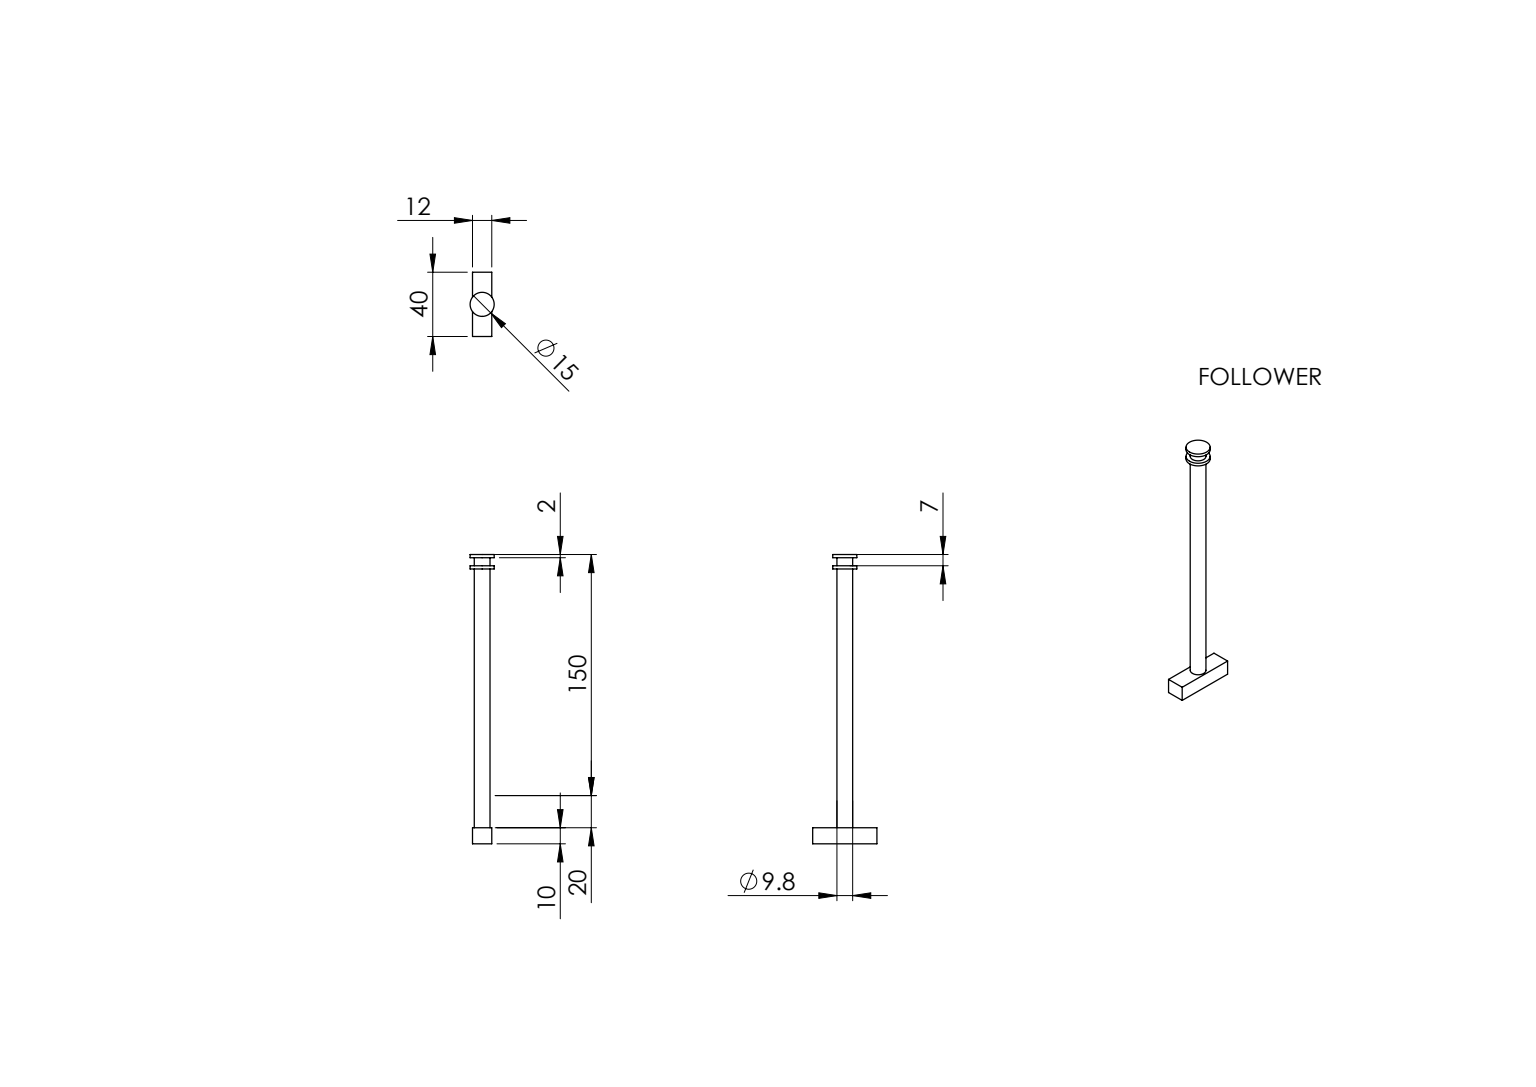
ISO-10303-21;
HEADER;
FILE_DESCRIPTION (('STEP AP214'),
    '1' );
FILE_NAME ('follower.step',
    '2026-10-31T03:36:27',
    ( '' ),
    ( '' ),
    'SwSTEP 2.0',
    'SolidWorks 2026',
    '' );
FILE_SCHEMA (( 'AUTOMOTIVE_DESIGN' ));
ENDSEC;

DATA;
#15=ORIENTED_EDGE ( 'NONE', *, *, #13669, .F. ) ;
#100=DIRECTION ( 'NONE',  ( -1.000000000000000000, 0.000000000000000000, 5.782411586589356653E-16 ) ) ;
#105=AXIS2_PLACEMENT_3D ( 'NONE', #31796, #37295, #28576 ) ;
#107=LINE ( 'NONE', #3514, #14620 ) ;
#160=UNCERTAINTY_MEASURE_WITH_UNIT (LENGTH_MEASURE( 1.000000000000000082E-05 ), #19760, 'distance_accuracy_value', 'NONE');
#194=CARTESIAN_POINT ( 'NONE',  ( 5.999999999999999112, -30.00000000000000000, -19.99999999999999289 ) ) ;
#273=FACE_OUTER_BOUND ( 'NONE', #13038, .T. ) ;
#337=AXIS2_PLACEMENT_3D ( 'NONE', #15365, #24083, #35628 ) ;
#423=CARTESIAN_POINT ( 'NONE',  ( 0.000000000000000000, 143.0000000000000000, 0.000000000000000000 ) ) ;
#429=ORIENTED_EDGE ( 'NONE', *, *, #547, .F. ) ;
#505=EDGE_LOOP ( 'NONE', ( #36598, #28782, #25690, #21960 ) ) ;
#547=EDGE_CURVE ( 'NONE', #14469, #8607, #31068, .T. ) ;
#642=CYLINDRICAL_SURFACE ( 'NONE', #12591, 4.899999999999999467 ) ;
#732=LINE ( 'NONE', #35796, #24881 ) ;
#762=VERTEX_POINT ( 'NONE', #1446 ) ;
#937=AXIS2_PLACEMENT_3D ( 'NONE', #24457, #33914, #7396 ) ;
#980=ORIENTED_EDGE ( 'NONE', *, *, #3451, .T. ) ;
#1025=ORIENTED_EDGE ( 'NONE', *, *, #37375, .T. ) ;
#1100=VECTOR ( 'NONE', #32793, 1000.000000000000000 ) ;
#1108=PLANE ( 'NONE',  #11917 ) ;
#1181=ORIENTED_EDGE ( 'NONE', *, *, #19610, .T. ) ;
#1231=ORIENTED_EDGE ( 'NONE', *, *, #34414, .F. ) ;
#1293=ADVANCED_FACE ( 'NONE', ( #273 ), #642, .T. ) ;
#1351=VERTEX_POINT ( 'NONE', #6531 ) ;
#1446=CARTESIAN_POINT ( 'NONE',  ( -6.000000000000000888, -30.00000000000000000, 20.00000000000000711 ) ) ;
#1468=LINE ( 'NONE', #22824, #18170 ) ;
#1631=SHAPE_DEFINITION_REPRESENTATION ( #19546, #8404 ) ;
#1734=VECTOR ( 'NONE', #11519, 1000.000000000000000 ) ;
#1890=ORIENTED_EDGE ( 'NONE', *, *, #32981, .F. ) ;
#2042=AXIS2_PLACEMENT_3D ( 'NONE', #31159, #28304, #16756 ) ;
#2104=CARTESIAN_POINT ( 'NONE',  ( 0.000000000000000000, 150.0000000000000000, 0.000000000000000000 ) ) ;
#2125=ORIENTED_EDGE ( 'NONE', *, *, #27701, .F. ) ;
#2222=EDGE_CURVE ( 'NONE', #13040, #5701, #9847, .T. ) ;
#2244=DIRECTION ( 'NONE',  ( 0.000000000000000000, 0.000000000000000000, 1.000000000000000000 ) ) ;
#2290=DIRECTION ( 'NONE',  ( 0.000000000000000000, -0.000000000000000000, 1.000000000000000000 ) ) ;
#2448=MECHANICAL_DESIGN_GEOMETRIC_PRESENTATION_REPRESENTATION('',(#13958),#24243);
#2589=DIRECTION ( 'NONE',  ( 0.000000000000000000, 0.000000000000000000, 1.000000000000000000 ) ) ;
#2592=ORIENTED_EDGE ( 'NONE', *, *, #17340, .F. ) ;
#2619=ORIENTED_EDGE ( 'NONE', *, *, #17340, .T. ) ;
#2703=PLANE ( 'NONE',  #2042 ) ;
#2990=CARTESIAN_POINT ( 'NONE',  ( 6.000000000000000000, -30.00000000000000000, 20.00000000000000000 ) ) ;
#3152=PRODUCT_DEFINITION_CONTEXT ( 'detailed design', #6891, 'design' ) ;
#3165=ORIENTED_EDGE ( 'NONE', *, *, #32431, .T. ) ;
#3269=CARTESIAN_POINT ( 'NONE',  ( 5.999999999999999112, -20.00000000000000000, -19.99999999999999289 ) ) ;
#3315=ADVANCED_FACE ( 'NONE', ( #19149 ), #27843, .T. ) ;
#3355=ORIENTED_EDGE ( 'NONE', *, *, #23085, .F. ) ;
#3361=ORIENTED_EDGE ( 'NONE', *, *, #26146, .F. ) ;
#3451=EDGE_CURVE ( 'NONE', #34986, #25827, #27661, .T. ) ;
#3459=EDGE_CURVE ( 'NONE', #4369, #32041, #34461, .T. ) ;
#3496=APPLICATION_CONTEXT ( 'automotive_design' ) ;
#3514=CARTESIAN_POINT ( 'NONE',  ( 6.000769315822030740E-16, -20.00000000000000000, -4.899999999999999467 ) ) ;
#3572=EDGE_CURVE ( 'NONE', #1351, #25827, #28567, .T. ) ;
#3716=DIRECTION ( 'NONE',  ( -1.000000000000000000, -0.000000000000000000, 5.782411586589356653E-16 ) ) ;
#3876=DIRECTION ( 'NONE',  ( 0.000000000000000000, 1.000000000000000000, 0.000000000000000000 ) ) ;
#3931=CARTESIAN_POINT ( 'NONE',  ( 0.000000000000000000, -20.00000000000000000, 0.000000000000000000 ) ) ;
#4270=EDGE_LOOP ( 'NONE', ( #13366, #36759, #31537, #32986 ) ) ;
#4310=ORIENTED_EDGE ( 'NONE', *, *, #8311, .F. ) ;
#4369=VERTEX_POINT ( 'NONE', #27616 ) ;
#4439=CARTESIAN_POINT ( 'NONE',  ( 0.000000000000000000, -20.00000000000000000, 4.899999999999999467 ) ) ;
#4528=DIRECTION ( 'NONE',  ( -0.000000000000000000, -1.000000000000000000, -0.000000000000000000 ) ) ;
#4534=DIRECTION ( 'NONE',  ( 0.000000000000000000, 1.000000000000000000, 0.000000000000000000 ) ) ;
#4651=DIRECTION ( 'NONE',  ( 0.000000000000000000, 0.000000000000000000, 1.000000000000000000 ) ) ;
#4744=CLOSED_SHELL ( 'NONE', ( #24245, #27494, #28200, #19192, #1293, #6469, #32100, #16308, #5411, #18285, #28238, #3315, #20115, #18072, #18295, #24769, #16663, #12725 ) ) ;
#4791=DIRECTION ( 'NONE',  ( 1.000000000000000000, 0.000000000000000000, -0.000000000000000000 ) ) ;
#4965=EDGE_CURVE ( 'NONE', #23915, #23913, #20695, .T. ) ;
#5029=AXIS2_PLACEMENT_3D ( 'NONE', #14926, #6766, #29888 ) ;
#5066=ORIENTED_EDGE ( 'NONE', *, *, #29640, .T. ) ;
#5156=AXIS2_PLACEMENT_3D ( 'NONE', #20310, #31851, #28999 ) ;
#5411=ADVANCED_FACE ( 'NONE', ( #19800 ), #2703, .F. ) ;
#5574=( NAMED_UNIT ( * ) SI_UNIT ( $, .STERADIAN. ) SOLID_ANGLE_UNIT ( ) );
#5638=( GEOMETRIC_REPRESENTATION_CONTEXT ( 3 ) GLOBAL_UNCERTAINTY_ASSIGNED_CONTEXT ( ( #13508 ) ) GLOBAL_UNIT_ASSIGNED_CONTEXT ( ( #28887, #11461, #29253 ) ) REPRESENTATION_CONTEXT ( 'NONE', 'WORKASPACE' ) );
#5701=VERTEX_POINT ( 'NONE', #3269 ) ;
#5922=DIRECTION ( 'NONE',  ( 0.000000000000000000, 1.000000000000000000, 0.000000000000000000 ) ) ;
#6136=( LENGTH_UNIT ( ) NAMED_UNIT ( * ) SI_UNIT ( .MILLI., .METRE. ) );
#6216=ORIENTED_EDGE ( 'NONE', *, *, #17958, .F. ) ;
#6401=CARTESIAN_POINT ( 'NONE',  ( 0.000000000000000000, 141.0000000000000000, 0.000000000000000000 ) ) ;
#6414=CIRCLE ( 'NONE', #27599, 7.500000000000000000 ) ;
#6469=ADVANCED_FACE ( 'NONE', ( #35440 ), #32035, .F. ) ;
#6488=DIRECTION ( 'NONE',  ( -0.000000000000000000, 1.000000000000000000, 0.000000000000000000 ) ) ;
#6494=PLANE ( 'NONE',  #20020 ) ;
#6531=CARTESIAN_POINT ( 'NONE',  ( 0.000000000000000000, 143.0000000000000000, 7.500000000000000000 ) ) ;
#6588=DIRECTION ( 'NONE',  ( 0.000000000000000000, 0.000000000000000000, 1.000000000000000000 ) ) ;
#6687=DIRECTION ( 'NONE',  ( 0.000000000000000000, 0.000000000000000000, 1.000000000000000000 ) ) ;
#6766=DIRECTION ( 'NONE',  ( 0.000000000000000000, 1.000000000000000000, 0.000000000000000000 ) ) ;
#6806=CARTESIAN_POINT ( 'NONE',  ( 6.000769315822030740E-16, 143.0000000000000000, -4.899999999999999467 ) ) ;
#6891=APPLICATION_CONTEXT ( 'automotive_design' ) ;
#6892=ORIENTED_EDGE ( 'NONE', *, *, #36787, .F. ) ;
#7018=DIRECTION ( 'NONE',  ( -0.000000000000000000, 1.000000000000000000, -0.000000000000000000 ) ) ;
#7054=DIRECTION ( 'NONE',  ( 0.000000000000000000, -0.000000000000000000, 1.000000000000000000 ) ) ;
#7078=CARTESIAN_POINT ( 'NONE',  ( 0.000000000000000000, 143.0000000000000000, 0.000000000000000000 ) ) ;
#7149=CIRCLE ( 'NONE', #12598, 4.899999999999999467 ) ;
#7267=EDGE_LOOP ( 'NONE', ( #10105, #34010 ) ) ;
#7396=DIRECTION ( 'NONE',  ( 0.000000000000000000, 0.000000000000000000, 1.000000000000000000 ) ) ;
#7467=STYLED_ITEM ( 'NONE', ( #17344 ), #35907 ) ;
#7491=CARTESIAN_POINT ( 'NONE',  ( 5.999999999999999112, -30.00000000000000000, -19.99999999999999289 ) ) ;
#7496=VERTEX_POINT ( 'NONE', #25098 ) ;
#7648=CARTESIAN_POINT ( 'NONE',  ( -6.000000000000000888, -30.00000000000000000, -19.99999999999999289 ) ) ;
#7757=FACE_OUTER_BOUND ( 'NONE', #22189, .T. ) ;
#7768=EDGE_CURVE ( 'NONE', #762, #9915, #37023, .T. ) ;
#7985=DIRECTION ( 'NONE',  ( 0.000000000000000000, 1.000000000000000000, 0.000000000000000000 ) ) ;
#8054=CIRCLE ( 'NONE', #28598, 4.899999999999999467 ) ;
#8094=DIRECTION ( 'NONE',  ( 2.168404344971009176E-17, 0.000000000000000000, 1.000000000000000000 ) ) ;
#8181=CARTESIAN_POINT ( 'NONE',  ( 0.000000000000000000, 148.0000000000000000, 0.000000000000000000 ) ) ;
#8260=AXIS2_PLACEMENT_3D ( 'NONE', #19386, #30564, #22590 ) ;
#8276=LINE ( 'NONE', #22868, #22656 ) ;
#8311=EDGE_CURVE ( 'NONE', #5701, #32041, #8276, .T. ) ;
#8404=SHAPE_REPRESENTATION ( 'follower', ( #17215 ), #5638 ) ;
#8607=VERTEX_POINT ( 'NONE', #4439 ) ;
#8615=EDGE_CURVE ( 'NONE', #15843, #24049, #26284, .T. ) ;
#8642=FACE_OUTER_BOUND ( 'NONE', #20757, .T. ) ;
#8721=DIRECTION ( 'NONE',  ( 0.000000000000000000, 0.000000000000000000, 1.000000000000000000 ) ) ;
#8873=EDGE_LOOP ( 'NONE', ( #10245, #20263 ) ) ;
#9188=AXIS2_PLACEMENT_3D ( 'NONE', #9942, #9199, #26621 ) ;
#9199=DIRECTION ( 'NONE',  ( -0.000000000000000000, -1.000000000000000000, -0.000000000000000000 ) ) ;
#9236=EDGE_CURVE ( 'NONE', #25827, #1351, #25523, .T. ) ;
#9335=CARTESIAN_POINT ( 'NONE',  ( 0.000000000000000000, -30.00000000000000000, 0.000000000000000000 ) ) ;
#9359=ORIENTED_EDGE ( 'NONE', *, *, #23079, .F. ) ;
#9580=EDGE_LOOP ( 'NONE', ( #4310, #6892, #14299, #1890 ) ) ;
#9657=EDGE_CURVE ( 'NONE', #17309, #23915, #107, .T. ) ;
#9705=VECTOR ( 'NONE', #31157, 1000.000000000000000 ) ;
#9847=LINE ( 'NONE', #21424, #28518 ) ;
#9887=FACE_OUTER_BOUND ( 'NONE', #27859, .T. ) ;
#9915=VERTEX_POINT ( 'NONE', #19064 ) ;
#9942=CARTESIAN_POINT ( 'NONE',  ( 0.000000000000000000, 148.0000000000000000, 0.000000000000000000 ) ) ;
#9961=DIRECTION ( 'NONE',  ( -0.000000000000000000, 1.000000000000000000, -0.000000000000000000 ) ) ;
#9999=ORIENTED_EDGE ( 'NONE', *, *, #31251, .T. ) ;
#10072=CARTESIAN_POINT ( 'NONE',  ( 0.000000000000000000, 148.0000000000000000, 0.000000000000000000 ) ) ;
#10105=ORIENTED_EDGE ( 'NONE', *, *, #10824, .T. ) ;
#10245=ORIENTED_EDGE ( 'NONE', *, *, #3572, .T. ) ;
#10299=EDGE_CURVE ( 'NONE', #33635, #17895, #36290, .T. ) ;
#10546=VECTOR ( 'NONE', #23007, 1000.000000000000000 ) ;
#10630=ORIENTED_EDGE ( 'NONE', *, *, #26990, .F. ) ;
#10782=DIRECTION ( 'NONE',  ( 0.000000000000000000, 1.000000000000000000, 0.000000000000000000 ) ) ;
#10824=EDGE_CURVE ( 'NONE', #14417, #17309, #8054, .T. ) ;
#11198=DIRECTION ( 'NONE',  ( 0.000000000000000000, 0.000000000000000000, 1.000000000000000000 ) ) ;
#11199=ORIENTED_EDGE ( 'NONE', *, *, #23085, .T. ) ;
#11324=VECTOR ( 'NONE', #21602, 1000.000000000000000 ) ;
#11348=ORIENTED_EDGE ( 'NONE', *, *, #4965, .T. ) ;
#11397=AXIS2_PLACEMENT_3D ( 'NONE', #23983, #3876, #15638 ) ;
#11457=EDGE_CURVE ( 'NONE', #12783, #1351, #20440, .T. ) ;
#11461=( NAMED_UNIT ( * ) PLANE_ANGLE_UNIT ( ) SI_UNIT ( $, .RADIAN. ) );
#11497=ORIENTED_EDGE ( 'NONE', *, *, #4965, .F. ) ;
#11519=DIRECTION ( 'NONE',  ( 0.000000000000000000, 1.000000000000000000, 0.000000000000000000 ) ) ;
#11529=DIRECTION ( 'NONE',  ( 0.000000000000000000, 0.000000000000000000, 1.000000000000000000 ) ) ;
#11541=ORIENTED_EDGE ( 'NONE', *, *, #9657, .F. ) ;
#11599=CARTESIAN_POINT ( 'NONE',  ( 9.184850993605147944E-16, 148.0000000000000000, -7.500000000000000000 ) ) ;
#11837=DIRECTION ( 'NONE',  ( 0.000000000000000000, 1.000000000000000000, 0.000000000000000000 ) ) ;
#11917=AXIS2_PLACEMENT_3D ( 'NONE', #29729, #30116, #15908 ) ;
#12591=AXIS2_PLACEMENT_3D ( 'NONE', #20571, #11837, #17914 ) ;
#12598=AXIS2_PLACEMENT_3D ( 'NONE', #7078, #18831, #6687 ) ;
#12618=EDGE_LOOP ( 'NONE', ( #15709, #11497 ) ) ;
#12707=AXIS2_PLACEMENT_3D ( 'NONE', #2104, #22214, #2290 ) ;
#12725=ADVANCED_FACE ( 'NONE', ( #30413 ), #33067, .T. ) ;
#12782=AXIS2_PLACEMENT_3D ( 'NONE', #32821, #21095, #18634 ) ;
#12783=VERTEX_POINT ( 'NONE', #13162 ) ;
#12809=AXIS2_PLACEMENT_3D ( 'NONE', #423, #5922, #23561 ) ;
#12930=PLANE ( 'NONE',  #26627 ) ;
#12936=CARTESIAN_POINT ( 'NONE',  ( 0.000000000000000000, 141.0000000000000000, 0.000000000000000000 ) ) ;
#13038=EDGE_LOOP ( 'NONE', ( #24183, #29294, #2619, #13486 ) ) ;
#13040=VERTEX_POINT ( 'NONE', #194 ) ;
#13162=CARTESIAN_POINT ( 'NONE',  ( 0.000000000000000000, 141.0000000000000000, 7.500000000000000000 ) ) ;
#13295=ORIENTED_EDGE ( 'NONE', *, *, #33728, .F. ) ;
#13366=ORIENTED_EDGE ( 'NONE', *, *, #8311, .T. ) ;
#13462=ORIENTED_EDGE ( 'NONE', *, *, #3572, .F. ) ;
#13481=DIRECTION ( 'NONE',  ( 0.000000000000000000, 1.000000000000000000, 0.000000000000000000 ) ) ;
#13486=ORIENTED_EDGE ( 'NONE', *, *, #24306, .T. ) ;
#13508=UNCERTAINTY_MEASURE_WITH_UNIT (LENGTH_MEASURE( 1.000000000000000082E-05 ), #28887, 'distance_accuracy_value', 'NONE');
#13515=DIRECTION ( 'NONE',  ( -0.000000000000000000, 0.000000000000000000, -1.000000000000000000 ) ) ;
#13564=CIRCLE ( 'NONE', #36544, 7.500000000000000000 ) ;
#13589=EDGE_CURVE ( 'NONE', #29332, #31166, #22996, .T. ) ;
#13590=VECTOR ( 'NONE', #35076, 1000.000000000000000 ) ;
#13669=EDGE_CURVE ( 'NONE', #15843, #29332, #1468, .T. ) ;
#13712=PLANE ( 'NONE',  #33355 ) ;
#13741=AXIS2_PLACEMENT_3D ( 'NONE', #15717, #15337, #26890 ) ;
#13827=CARTESIAN_POINT ( 'NONE',  ( 6.000769315822030740E-16, 148.0000000000000000, -4.899999999999999467 ) ) ;
#13861=DIRECTION ( 'NONE',  ( -0.000000000000000000, -1.000000000000000000, -0.000000000000000000 ) ) ;
#13958=STYLED_ITEM('',(#37535),#20157);
#14134=ORIENTED_EDGE ( 'NONE', *, *, #10824, .F. ) ;
#14269=LINE ( 'NONE', #11599, #14305 ) ;
#14299=ORIENTED_EDGE ( 'NONE', *, *, #10299, .F. ) ;
#14305=VECTOR ( 'NONE', #23174, 1000.000000000000000 ) ;
#14417=VERTEX_POINT ( 'NONE', #35675 ) ;
#14469=VERTEX_POINT ( 'NONE', #18260 ) ;
#14553=CARTESIAN_POINT ( 'NONE',  ( 0.000000000000000000, 141.0000000000000000, 7.500000000000000000 ) ) ;
#14620=VECTOR ( 'NONE', #18123, 1000.000000000000000 ) ;
#14754=CARTESIAN_POINT ( 'NONE',  ( 9.184850993605147944E-16, 150.0000000000000000, -7.500000000000000000 ) ) ;
#14842=CARTESIAN_POINT ( 'NONE',  ( -6.000000000000000888, -20.00000000000000000, 20.00000000000000711 ) ) ;
#14926=CARTESIAN_POINT ( 'NONE',  ( 0.000000000000000000, -20.00000000000000000, 0.000000000000000000 ) ) ;
#15209=PLANE ( 'NONE',  #12707 ) ;
#15225=EDGE_LOOP ( 'NONE', ( #23468, #3355 ) ) ;
#15278=CARTESIAN_POINT ( 'NONE',  ( -6.000000000000000888, -30.00000000000000000, 20.00000000000000711 ) ) ;
#15286=CARTESIAN_POINT ( 'NONE',  ( 0.000000000000000000, 148.0000000000000000, 7.500000000000000000 ) ) ;
#15337=DIRECTION ( 'NONE',  ( 0.000000000000000000, 1.000000000000000000, 0.000000000000000000 ) ) ;
#15365=CARTESIAN_POINT ( 'NONE',  ( 5.999999999999999112, -30.00000000000000000, -19.99999999999999289 ) ) ;
#15367=LINE ( 'NONE', #15555, #1100 ) ;
#15528=FACE_BOUND ( 'NONE', #22217, .T. ) ;
#15555=CARTESIAN_POINT ( 'NONE',  ( -6.000000000000000888, -30.00000000000000000, -19.99999999999999289 ) ) ;
#15638=DIRECTION ( 'NONE',  ( 0.000000000000000000, 0.000000000000000000, 1.000000000000000000 ) ) ;
#15698=ORIENTED_EDGE ( 'NONE', *, *, #19610, .F. ) ;
#15709=ORIENTED_EDGE ( 'NONE', *, *, #21328, .F. ) ;
#15717=CARTESIAN_POINT ( 'NONE',  ( 0.000000000000000000, 141.0000000000000000, 0.000000000000000000 ) ) ;
#15786=FACE_OUTER_BOUND ( 'NONE', #15225, .T. ) ;
#15821=ORIENTED_EDGE ( 'NONE', *, *, #13589, .T. ) ;
#15843=VERTEX_POINT ( 'NONE', #15286 ) ;
#15846=CARTESIAN_POINT ( 'NONE',  ( -6.000000000000000888, -20.00000000000000000, -19.99999999999999289 ) ) ;
#15887=EDGE_LOOP ( 'NONE', ( #1025, #980, #13462, #33477 ) ) ;
#15908=DIRECTION ( 'NONE',  ( 0.000000000000000000, -0.000000000000000000, 1.000000000000000000 ) ) ;
#15941=EDGE_LOOP ( 'NONE', ( #13295, #30197, #11348, #9359 ) ) ;
#16047=CARTESIAN_POINT ( 'NONE',  ( 0.000000000000000000, 0.000000000000000000, 0.000000000000000000 ) ) ;
#16205=DIRECTION ( 'NONE',  ( 0.000000000000000000, 0.000000000000000000, 1.000000000000000000 ) ) ;
#16308=ADVANCED_FACE ( 'NONE', ( #33609 ), #13712, .F. ) ;
#16473=VECTOR ( 'NONE', #4534, 1000.000000000000000 ) ;
#16625=AXIS2_PLACEMENT_3D ( 'NONE', #6401, #34827, #6588 ) ;
#16663=ADVANCED_FACE ( 'NONE', ( #27319, #29781 ), #27510, .F. ) ;
#16673=CARTESIAN_POINT ( 'NONE',  ( 0.000000000000000000, 148.0000000000000000, 4.899999999999999467 ) ) ;
#16756=DIRECTION ( 'NONE',  ( 1.000000000000000000, 0.000000000000000000, 0.000000000000000000 ) ) ;
#16766=CIRCLE ( 'NONE', #34315, 4.899999999999999467 ) ;
#16872=EDGE_LOOP ( 'NONE', ( #11541, #14134, #20226, #17540 ) ) ;
#16902=( NAMED_UNIT ( * ) SI_UNIT ( $, .STERADIAN. ) SOLID_ANGLE_UNIT ( ) );
#17055=ORIENTED_EDGE ( 'NONE', *, *, #32981, .T. ) ;
#17159=SURFACE_STYLE_FILL_AREA ( #31367 ) ;
#17193=DIRECTION ( 'NONE',  ( 0.000000000000000000, 1.000000000000000000, 0.000000000000000000 ) ) ;
#17214=PRODUCT_DEFINITION_FORMATION_WITH_SPECIFIED_SOURCE ( 'ANY', '', #28601, .NOT_KNOWN. ) ;
#17215=AXIS2_PLACEMENT_3D ( 'NONE', #16047, #4651, #19645 ) ;
#17309=VERTEX_POINT ( 'NONE', #6806 ) ;
#17340=EDGE_CURVE ( 'NONE', #8607, #27046, #732, .T. ) ;
#17344=PRESENTATION_STYLE_ASSIGNMENT (( #23215 ) ) ;
#17361=CIRCLE ( 'NONE', #30073, 4.899999999999999467 ) ;
#17481=EDGE_CURVE ( 'NONE', #9915, #17895, #26639, .T. ) ;
#17507=ORIENTED_EDGE ( 'NONE', *, *, #24306, .F. ) ;
#17540=ORIENTED_EDGE ( 'NONE', *, *, #21328, .T. ) ;
#17569=ORIENTED_EDGE ( 'NONE', *, *, #8615, .F. ) ;
#17714=SHAPE_REPRESENTATION_RELATIONSHIP ( 'NONE' , 'NONE' ,  #8404, #35907 ) ;
#17755=( GEOMETRIC_REPRESENTATION_CONTEXT ( 3 ) GLOBAL_UNCERTAINTY_ASSIGNED_CONTEXT ( ( #36618 ) ) GLOBAL_UNIT_ASSIGNED_CONTEXT ( ( #6136, #34764, #5574 ) ) REPRESENTATION_CONTEXT ( 'NONE', 'WORKASPACE' ) );
#17895=VERTEX_POINT ( 'NONE', #27393 ) ;
#17914=DIRECTION ( 'NONE',  ( 0.000000000000000000, 0.000000000000000000, 1.000000000000000000 ) ) ;
#17927=CARTESIAN_POINT ( 'NONE',  ( 6.000000000000000000, -20.00000000000000000, 20.00000000000000000 ) ) ;
#17958=EDGE_CURVE ( 'NONE', #762, #33635, #30244, .T. ) ;
#18068=DIRECTION ( 'NONE',  ( 0.000000000000000000, 1.000000000000000000, 0.000000000000000000 ) ) ;
#18072=ADVANCED_FACE ( 'NONE', ( #36039, #21652 ), #35662, .T. ) ;
#18123=DIRECTION ( 'NONE',  ( 0.000000000000000000, 1.000000000000000000, 0.000000000000000000 ) ) ;
#18170=VECTOR ( 'NONE', #37207, 1000.000000000000000 ) ;
#18248=FACE_OUTER_BOUND ( 'NONE', #34451, .T. ) ;
#18260=CARTESIAN_POINT ( 'NONE',  ( 6.000769315822030740E-16, -20.00000000000000000, -4.899999999999999467 ) ) ;
#18273=EDGE_LOOP ( 'NONE', ( #17507, #19442 ) ) ;
#18285=ADVANCED_FACE ( 'NONE', ( #18820 ), #12930, .F. ) ;
#18295=ADVANCED_FACE ( 'NONE', ( #18248 ), #15209, .T. ) ;
#18358=DIRECTION ( 'NONE',  ( 0.000000000000000000, 1.000000000000000000, 0.000000000000000000 ) ) ;
#18634=DIRECTION ( 'NONE',  ( 0.000000000000000000, -0.000000000000000000, 1.000000000000000000 ) ) ;
#18697=LINE ( 'NONE', #7491, #21451 ) ;
#18820=FACE_OUTER_BOUND ( 'NONE', #28924, .T. ) ;
#18831=DIRECTION ( 'NONE',  ( -0.000000000000000000, -1.000000000000000000, -0.000000000000000000 ) ) ;
#19064=CARTESIAN_POINT ( 'NONE',  ( -6.000000000000000888, -30.00000000000000000, -19.99999999999999289 ) ) ;
#19098=AXIS2_PLACEMENT_3D ( 'NONE', #34610, #17193, #2589 ) ;
#19149=FACE_OUTER_BOUND ( 'NONE', #31266, .T. ) ;
#19192=ADVANCED_FACE ( 'NONE', ( #7757 ), #24811, .T. ) ;
#19386=CARTESIAN_POINT ( 'NONE',  ( 0.000000000000000000, 148.0000000000000000, 0.000000000000000000 ) ) ;
#19442=ORIENTED_EDGE ( 'NONE', *, *, #27777, .F. ) ;
#19546=PRODUCT_DEFINITION_SHAPE ( 'NONE', 'NONE',  #28710 ) ;
#19610=EDGE_CURVE ( 'NONE', #4369, #762, #31334, .T. ) ;
#19641=VECTOR ( 'NONE', #3716, 1000.000000000000000 ) ;
#19645=DIRECTION ( 'NONE',  ( 1.000000000000000000, 0.000000000000000000, 0.000000000000000000 ) ) ;
#19760=( LENGTH_UNIT ( ) NAMED_UNIT ( * ) SI_UNIT ( .MILLI., .METRE. ) );
#19800=FACE_OUTER_BOUND ( 'NONE', #26486, .T. ) ;
#19892=DIRECTION ( 'NONE',  ( -0.000000000000000000, 1.000000000000000000, -0.000000000000000000 ) ) ;
#19959=CARTESIAN_POINT ( 'NONE',  ( 0.000000000000000000, 150.0000000000000000, 7.500000000000000000 ) ) ;
#20020=AXIS2_PLACEMENT_3D ( 'NONE', #12936, #18068, #21103 ) ;
#20045=DIRECTION ( 'NONE',  ( -0.000000000000000000, 1.000000000000000000, -0.000000000000000000 ) ) ;
#20115=ADVANCED_FACE ( 'NONE', ( #35479, #15786 ), #6494, .F. ) ;
#20157=MANIFOLD_SOLID_BREP ( 'LPattern2', #4744 ) ;
#20226=ORIENTED_EDGE ( 'NONE', *, *, #23079, .T. ) ;
#20263=ORIENTED_EDGE ( 'NONE', *, *, #9236, .T. ) ;
#20310=CARTESIAN_POINT ( 'NONE',  ( 0.000000000000000000, 141.0000000000000000, 0.000000000000000000 ) ) ;
#20372=AXIS2_PLACEMENT_3D ( 'NONE', #22211, #13481, #25035 ) ;
#20440=LINE ( 'NONE', #14553, #1734 ) ;
#20571=CARTESIAN_POINT ( 'NONE',  ( 0.000000000000000000, -20.00000000000000000, 0.000000000000000000 ) ) ;
#20695=CIRCLE ( 'NONE', #9188, 4.899999999999999467 ) ;
#20757=EDGE_LOOP ( 'NONE', ( #17055, #6216, #15698, #33758 ) ) ;
#21014=CARTESIAN_POINT ( 'NONE',  ( 9.184850993605147944E-16, 148.0000000000000000, -7.500000000000000000 ) ) ;
#21015=DIRECTION ( 'NONE',  ( 0.000000000000000000, 1.000000000000000000, 0.000000000000000000 ) ) ;
#21095=DIRECTION ( 'NONE',  ( 0.000000000000000000, 1.000000000000000000, 0.000000000000000000 ) ) ;
#21103=DIRECTION ( 'NONE',  ( 0.000000000000000000, -0.000000000000000000, 1.000000000000000000 ) ) ;
#21121=ORIENTED_EDGE ( 'NONE', *, *, #36787, .T. ) ;
#21154=ORIENTED_EDGE ( 'NONE', *, *, #2222, .F. ) ;
#21328=EDGE_CURVE ( 'NONE', #23913, #23915, #27632, .T. ) ;
#21393=MECHANICAL_DESIGN_GEOMETRIC_PRESENTATION_REPRESENTATION('',(#7467),#17755);
#21424=CARTESIAN_POINT ( 'NONE',  ( 5.999999999999999112, -30.00000000000000000, -19.99999999999999289 ) ) ;
#21451=VECTOR ( 'NONE', #30047, 1000.000000000000000 ) ;
#21518=ORIENTED_EDGE ( 'NONE', *, *, #31251, .F. ) ;
#21575=CYLINDRICAL_SURFACE ( 'NONE', #34224, 4.899999999999999467 ) ;
#21602=DIRECTION ( 'NONE',  ( 0.000000000000000000, 1.000000000000000000, 0.000000000000000000 ) ) ;
#21652=FACE_OUTER_BOUND ( 'NONE', #8873, .T. ) ;
#21782=CYLINDRICAL_SURFACE ( 'NONE', #13741, 7.500000000000000000 ) ;
#21791=DIRECTION ( 'NONE',  ( 0.000000000000000000, 0.000000000000000000, 1.000000000000000000 ) ) ;
#21937=AXIS2_PLACEMENT_3D ( 'NONE', #25556, #10782, #24813 ) ;
#21951=EDGE_LOOP ( 'NONE', ( #10630, #29764, #35685, #21518 ) ) ;
#21960=ORIENTED_EDGE ( 'NONE', *, *, #17958, .T. ) ;
#21985=DIRECTION ( 'NONE',  ( 0.000000000000000000, 1.000000000000000000, 0.000000000000000000 ) ) ;
#21991=ORIENTED_EDGE ( 'NONE', *, *, #8615, .T. ) ;
#22189=EDGE_LOOP ( 'NONE', ( #24463, #5066, #32610, #2592 ) ) ;
#22211=CARTESIAN_POINT ( 'NONE',  ( 0.000000000000000000, 148.0000000000000000, 0.000000000000000000 ) ) ;
#22214=DIRECTION ( 'NONE',  ( 0.000000000000000000, 1.000000000000000000, 0.000000000000000000 ) ) ;
#22217=EDGE_LOOP ( 'NONE', ( #2125, #429 ) ) ;
#22484=VECTOR ( 'NONE', #9961, 1000.000000000000000 ) ;
#22590=DIRECTION ( 'NONE',  ( 0.000000000000000000, 0.000000000000000000, 1.000000000000000000 ) ) ;
#22656=VECTOR ( 'NONE', #8094, 1000.000000000000000 ) ;
#22824=CARTESIAN_POINT ( 'NONE',  ( 0.000000000000000000, 148.0000000000000000, 7.500000000000000000 ) ) ;
#22868=CARTESIAN_POINT ( 'NONE',  ( 5.999999999999999112, -20.00000000000000000, -19.99999999999999289 ) ) ;
#22996=CIRCLE ( 'NONE', #33902, 7.500000000000000000 ) ;
#23007=DIRECTION ( 'NONE',  ( -0.000000000000000000, -0.000000000000000000, -1.000000000000000000 ) ) ;
#23079=EDGE_CURVE ( 'NONE', #14417, #23913, #25528, .T. ) ;
#23085=EDGE_CURVE ( 'NONE', #34986, #12783, #33607, .T. ) ;
#23174=DIRECTION ( 'NONE',  ( 0.000000000000000000, 1.000000000000000000, 0.000000000000000000 ) ) ;
#23215=SURFACE_STYLE_USAGE ( .BOTH. , #25680 ) ;
#23468=ORIENTED_EDGE ( 'NONE', *, *, #37375, .F. ) ;
#23561=DIRECTION ( 'NONE',  ( 0.000000000000000000, 0.000000000000000000, 1.000000000000000000 ) ) ;
#23913=VERTEX_POINT ( 'NONE', #16673 ) ;
#23915=VERTEX_POINT ( 'NONE', #13827 ) ;
#23983=CARTESIAN_POINT ( 'NONE',  ( 0.000000000000000000, -20.00000000000000000, 0.000000000000000000 ) ) ;
#24049=VERTEX_POINT ( 'NONE', #21014 ) ;
#24083=DIRECTION ( 'NONE',  ( -1.000000000000000000, 0.000000000000000000, 2.168404344971009484E-17 ) ) ;
#24183=ORIENTED_EDGE ( 'NONE', *, *, #29640, .F. ) ;
#24211=AXIS2_PLACEMENT_3D ( 'NONE', #36362, #21985, #2244 ) ;
#24220=FACE_OUTER_BOUND ( 'NONE', #15941, .T. ) ;
#24243=( GEOMETRIC_REPRESENTATION_CONTEXT ( 3 ) GLOBAL_UNCERTAINTY_ASSIGNED_CONTEXT ( ( #160 ) ) GLOBAL_UNIT_ASSIGNED_CONTEXT ( ( #19760, #28076, #16902 ) ) REPRESENTATION_CONTEXT ( 'NONE', 'WORKASPACE' ) );
#24245=ADVANCED_FACE ( 'NONE', ( #24220 ), #21575, .T. ) ;
#24297=DIRECTION ( 'NONE',  ( 0.000000000000000000, 1.000000000000000000, 0.000000000000000000 ) ) ;
#24306=EDGE_CURVE ( 'NONE', #27046, #7496, #26943, .T. ) ;
#24414=COLOUR_RGB ( '',0.8941176470588234615, 0.8941176470588234615, 0.8941176470588234615 ) ;
#24457=CARTESIAN_POINT ( 'NONE',  ( 0.000000000000000000, 148.0000000000000000, 0.000000000000000000 ) ) ;
#24463=ORIENTED_EDGE ( 'NONE', *, *, #27701, .T. ) ;
#24539=DIRECTION ( 'NONE',  ( 0.000000000000000000, 1.000000000000000000, 0.000000000000000000 ) ) ;
#24769=ADVANCED_FACE ( 'NONE', ( #36188 ), #33542, .T. ) ;
#24811=CYLINDRICAL_SURFACE ( 'NONE', #24211, 4.899999999999999467 ) ;
#24813=DIRECTION ( 'NONE',  ( 0.000000000000000000, 0.000000000000000000, 1.000000000000000000 ) ) ;
#24881=VECTOR ( 'NONE', #29550, 1000.000000000000000 ) ;
#25035=DIRECTION ( 'NONE',  ( 0.000000000000000000, 0.000000000000000000, 1.000000000000000000 ) ) ;
#25098=CARTESIAN_POINT ( 'NONE',  ( 6.000769315822030740E-16, 141.0000000000000000, -4.899999999999999467 ) ) ;
#25152=ORIENTED_EDGE ( 'NONE', *, *, #13589, .F. ) ;
#25523=CIRCLE ( 'NONE', #12809, 7.500000000000000000 ) ;
#25528=LINE ( 'NONE', #34248, #28162 ) ;
#25556=CARTESIAN_POINT ( 'NONE',  ( 0.000000000000000000, 141.0000000000000000, 0.000000000000000000 ) ) ;
#25632=CARTESIAN_POINT ( 'NONE',  ( 0.000000000000000000, 141.0000000000000000, 4.899999999999999467 ) ) ;
#25671=LINE ( 'NONE', #32237, #13590 ) ;
#25680=SURFACE_SIDE_STYLE ('',( #17159 ) ) ;
#25690=ORIENTED_EDGE ( 'NONE', *, *, #7768, .F. ) ;
#25827=VERTEX_POINT ( 'NONE', #34571 ) ;
#26072=DIRECTION ( 'NONE',  ( -5.782411586589356653E-16, 0.000000000000000000, -1.000000000000000000 ) ) ;
#26146=EDGE_CURVE ( 'NONE', #24049, #15843, #6414, .T. ) ;
#26284=CIRCLE ( 'NONE', #34161, 7.500000000000000000 ) ;
#26486=EDGE_LOOP ( 'NONE', ( #21121, #21154, #1231, #34359 ) ) ;
#26621=DIRECTION ( 'NONE',  ( 0.000000000000000000, 0.000000000000000000, 1.000000000000000000 ) ) ;
#26627=AXIS2_PLACEMENT_3D ( 'NONE', #9335, #6488, #29603 ) ;
#26639=LINE ( 'NONE', #32331, #29720 ) ;
#26678=DIRECTION ( 'NONE',  ( 0.000000000000000000, 0.000000000000000000, 1.000000000000000000 ) ) ;
#26890=DIRECTION ( 'NONE',  ( 0.000000000000000000, 0.000000000000000000, 1.000000000000000000 ) ) ;
#26943=CIRCLE ( 'NONE', #5156, 4.899999999999999467 ) ;
#26990=EDGE_CURVE ( 'NONE', #24049, #31166, #14269, .T. ) ;
#27046=VERTEX_POINT ( 'NONE', #25632 ) ;
#27089=CARTESIAN_POINT ( 'NONE',  ( 6.000769315822030740E-16, -20.00000000000000000, -4.899999999999999467 ) ) ;
#27191=CARTESIAN_POINT ( 'NONE',  ( 0.000000000000000000, 148.0000000000000000, 0.000000000000000000 ) ) ;
#27319=FACE_BOUND ( 'NONE', #12618, .T. ) ;
#27393=CARTESIAN_POINT ( 'NONE',  ( -6.000000000000000888, -20.00000000000000000, -19.99999999999999289 ) ) ;
#27415=VECTOR ( 'NONE', #33457, 1000.000000000000000 ) ;
#27433=ORIENTED_EDGE ( 'NONE', *, *, #11457, .T. ) ;
#27466=CARTESIAN_POINT ( 'NONE',  ( 0.000000000000000000, 143.0000000000000000, 0.000000000000000000 ) ) ;
#27494=ADVANCED_FACE ( 'NONE', ( #9887 ), #33010, .T. ) ;
#27510=PLANE ( 'NONE',  #35781 ) ;
#27599=AXIS2_PLACEMENT_3D ( 'NONE', #8181, #31658, #11198 ) ;
#27616=CARTESIAN_POINT ( 'NONE',  ( 6.000000000000000000, -30.00000000000000000, 20.00000000000000000 ) ) ;
#27632=CIRCLE ( 'NONE', #8260, 4.899999999999999467 ) ;
#27661=LINE ( 'NONE', #30514, #16473 ) ;
#27701=EDGE_CURVE ( 'NONE', #8607, #14469, #16766, .T. ) ;
#27777=EDGE_CURVE ( 'NONE', #7496, #27046, #17361, .T. ) ;
#27843=CYLINDRICAL_SURFACE ( 'NONE', #21937, 7.500000000000000000 ) ;
#27852=CARTESIAN_POINT ( 'NONE',  ( 9.184850993605147944E-16, 141.0000000000000000, -7.500000000000000000 ) ) ;
#27859=EDGE_LOOP ( 'NONE', ( #21991, #34555, #25152, #15 ) ) ;
#28076=( NAMED_UNIT ( * ) PLANE_ANGLE_UNIT ( ) SI_UNIT ( $, .RADIAN. ) );
#28082=AXIS2_PLACEMENT_3D ( 'NONE', #28910, #26072, #100 ) ;
#28117=CARTESIAN_POINT ( 'NONE',  ( -6.000000000000000888, -30.00000000000000000, 20.00000000000000711 ) ) ;
#28162=VECTOR ( 'NONE', #31220, 1000.000000000000000 ) ;
#28200=ADVANCED_FACE ( 'NONE', ( #29924 ), #21782, .T. ) ;
#28238=ADVANCED_FACE ( 'NONE', ( #15528, #29544 ), #1108, .T. ) ;
#28255=CARTESIAN_POINT ( 'NONE',  ( 0.000000000000000000, 141.0000000000000000, 0.000000000000000000 ) ) ;
#28304=DIRECTION ( 'NONE',  ( -0.000000000000000000, 0.000000000000000000, 1.000000000000000000 ) ) ;
#28518=VECTOR ( 'NONE', #7018, 1000.000000000000000 ) ;
#28567=CIRCLE ( 'NONE', #105, 7.500000000000000000 ) ;
#28576=DIRECTION ( 'NONE',  ( 0.000000000000000000, 0.000000000000000000, 1.000000000000000000 ) ) ;
#28598=AXIS2_PLACEMENT_3D ( 'NONE', #27466, #4528, #21791 ) ;
#28601=PRODUCT ( 'follower', 'follower', '', ( #32908 ) ) ;
#28710=PRODUCT_DEFINITION ( 'UNKNOWN', '', #17214, #3152 ) ;
#28782=ORIENTED_EDGE ( 'NONE', *, *, #17481, .F. ) ;
#28887=( LENGTH_UNIT ( ) NAMED_UNIT ( * ) SI_UNIT ( .MILLI., .METRE. ) );
#28910=CARTESIAN_POINT ( 'NONE',  ( -6.000000000000000888, -30.00000000000000000, 20.00000000000000711 ) ) ;
#28924=EDGE_LOOP ( 'NONE', ( #3165, #1181, #30336, #30179 ) ) ;
#28999=DIRECTION ( 'NONE',  ( 0.000000000000000000, 0.000000000000000000, 1.000000000000000000 ) ) ;
#29253=( NAMED_UNIT ( * ) SI_UNIT ( $, .STERADIAN. ) SOLID_ANGLE_UNIT ( ) );
#29294=ORIENTED_EDGE ( 'NONE', *, *, #547, .T. ) ;
#29332=VERTEX_POINT ( 'NONE', #19959 ) ;
#29335=CARTESIAN_POINT ( 'NONE',  ( 0.000000000000000000, 150.0000000000000000, 0.000000000000000000 ) ) ;
#29544=FACE_OUTER_BOUND ( 'NONE', #9580, .T. ) ;
#29550=DIRECTION ( 'NONE',  ( 0.000000000000000000, 1.000000000000000000, 0.000000000000000000 ) ) ;
#29603=DIRECTION ( 'NONE',  ( 0.000000000000000000, -0.000000000000000000, 1.000000000000000000 ) ) ;
#29640=EDGE_CURVE ( 'NONE', #14469, #7496, #33338, .T. ) ;
#29682=CARTESIAN_POINT ( 'NONE',  ( -6.000000000000000888, -20.00000000000000000, 20.00000000000000711 ) ) ;
#29720=VECTOR ( 'NONE', #20045, 1000.000000000000000 ) ;
#29729=CARTESIAN_POINT ( 'NONE',  ( 0.000000000000000000, -20.00000000000000000, 0.000000000000000000 ) ) ;
#29764=ORIENTED_EDGE ( 'NONE', *, *, #26146, .T. ) ;
#29781=FACE_OUTER_BOUND ( 'NONE', #37399, .T. ) ;
#29807=ORIENTED_EDGE ( 'NONE', *, *, #3451, .F. ) ;
#29888=DIRECTION ( 'NONE',  ( 0.000000000000000000, 0.000000000000000000, 1.000000000000000000 ) ) ;
#29924=FACE_OUTER_BOUND ( 'NONE', #15887, .T. ) ;
#30047=DIRECTION ( 'NONE',  ( 2.168404344971009176E-17, 0.000000000000000000, 1.000000000000000000 ) ) ;
#30073=AXIS2_PLACEMENT_3D ( 'NONE', #28255, #13861, #31287 ) ;
#30090=DIRECTION ( 'NONE',  ( 0.000000000000000000, 1.000000000000000000, 0.000000000000000000 ) ) ;
#30116=DIRECTION ( 'NONE',  ( -0.000000000000000000, 1.000000000000000000, 0.000000000000000000 ) ) ;
#30179=ORIENTED_EDGE ( 'NONE', *, *, #34414, .T. ) ;
#30197=ORIENTED_EDGE ( 'NONE', *, *, #9657, .T. ) ;
#30244=LINE ( 'NONE', #15278, #22484 ) ;
#30336=ORIENTED_EDGE ( 'NONE', *, *, #7768, .T. ) ;
#30413=FACE_OUTER_BOUND ( 'NONE', #16872, .T. ) ;
#30514=CARTESIAN_POINT ( 'NONE',  ( 9.184850993605147944E-16, 141.0000000000000000, -7.500000000000000000 ) ) ;
#30564=DIRECTION ( 'NONE',  ( -0.000000000000000000, -1.000000000000000000, -0.000000000000000000 ) ) ;
#31068=CIRCLE ( 'NONE', #5029, 4.899999999999999467 ) ;
#31157=DIRECTION ( 'NONE',  ( -1.000000000000000000, -0.000000000000000000, 5.782411586589356653E-16 ) ) ;
#31159=CARTESIAN_POINT ( 'NONE',  ( -6.000000000000000888, -30.00000000000000000, -19.99999999999999289 ) ) ;
#31166=VERTEX_POINT ( 'NONE', #14754 ) ;
#31220=DIRECTION ( 'NONE',  ( 0.000000000000000000, 1.000000000000000000, 0.000000000000000000 ) ) ;
#31251=EDGE_CURVE ( 'NONE', #31166, #29332, #13564, .T. ) ;
#31266=EDGE_LOOP ( 'NONE', ( #29807, #11199, #27433, #31844 ) ) ;
#31287=DIRECTION ( 'NONE',  ( 0.000000000000000000, 0.000000000000000000, 1.000000000000000000 ) ) ;
#31334=LINE ( 'NONE', #28117, #9705 ) ;
#31367=FILL_AREA_STYLE ('',( #31550 ) ) ;
#31537=ORIENTED_EDGE ( 'NONE', *, *, #32431, .F. ) ;
#31550=FILL_AREA_STYLE_COLOUR ( '', #24414 ) ;
#31658=DIRECTION ( 'NONE',  ( 0.000000000000000000, 1.000000000000000000, 0.000000000000000000 ) ) ;
#31759=PLANE ( 'NONE',  #28082 ) ;
#31796=CARTESIAN_POINT ( 'NONE',  ( 0.000000000000000000, 143.0000000000000000, 0.000000000000000000 ) ) ;
#31844=ORIENTED_EDGE ( 'NONE', *, *, #9236, .F. ) ;
#31851=DIRECTION ( 'NONE',  ( -0.000000000000000000, -1.000000000000000000, -0.000000000000000000 ) ) ;
#32035=PLANE ( 'NONE',  #337 ) ;
#32041=VERTEX_POINT ( 'NONE', #17927 ) ;
#32100=ADVANCED_FACE ( 'NONE', ( #8642 ), #31759, .F. ) ;
#32237=CARTESIAN_POINT ( 'NONE',  ( -6.000000000000000888, -20.00000000000000000, -19.99999999999999289 ) ) ;
#32331=CARTESIAN_POINT ( 'NONE',  ( -6.000000000000000888, -30.00000000000000000, -19.99999999999999289 ) ) ;
#32431=EDGE_CURVE ( 'NONE', #13040, #4369, #18697, .T. ) ;
#32522=LINE ( 'NONE', #29682, #19641 ) ;
#32610=ORIENTED_EDGE ( 'NONE', *, *, #27777, .T. ) ;
#32793=DIRECTION ( 'NONE',  ( 1.000000000000000000, 0.000000000000000000, 0.000000000000000000 ) ) ;
#32821=CARTESIAN_POINT ( 'NONE',  ( 0.000000000000000000, 143.0000000000000000, 0.000000000000000000 ) ) ;
#32908=PRODUCT_CONTEXT ( 'NONE', #3496, 'mechanical' ) ;
#32981=EDGE_CURVE ( 'NONE', #32041, #33635, #32522, .T. ) ;
#32986=ORIENTED_EDGE ( 'NONE', *, *, #2222, .T. ) ;
#33010=CYLINDRICAL_SURFACE ( 'NONE', #20372, 7.500000000000000000 ) ;
#33067=CYLINDRICAL_SURFACE ( 'NONE', #11397, 4.899999999999999467 ) ;
#33338=LINE ( 'NONE', #27089, #11324 ) ;
#33355=AXIS2_PLACEMENT_3D ( 'NONE', #7648, #4791, #13515 ) ;
#33457=DIRECTION ( 'NONE',  ( -0.000000000000000000, -0.000000000000000000, -1.000000000000000000 ) ) ;
#33477=ORIENTED_EDGE ( 'NONE', *, *, #11457, .F. ) ;
#33542=CYLINDRICAL_SURFACE ( 'NONE', #937, 7.500000000000000000 ) ;
#33607=CIRCLE ( 'NONE', #19098, 7.500000000000000000 ) ;
#33609=FACE_OUTER_BOUND ( 'NONE', #505, .T. ) ;
#33635=VERTEX_POINT ( 'NONE', #14842 ) ;
#33728=EDGE_CURVE ( 'NONE', #17309, #14417, #7149, .T. ) ;
#33758=ORIENTED_EDGE ( 'NONE', *, *, #3459, .T. ) ;
#33902=AXIS2_PLACEMENT_3D ( 'NONE', #29335, #18358, #26678 ) ;
#33914=DIRECTION ( 'NONE',  ( 0.000000000000000000, 1.000000000000000000, 0.000000000000000000 ) ) ;
#34010=ORIENTED_EDGE ( 'NONE', *, *, #33728, .T. ) ;
#34161=AXIS2_PLACEMENT_3D ( 'NONE', #27191, #24539, #16205 ) ;
#34224=AXIS2_PLACEMENT_3D ( 'NONE', #3931, #30090, #35766 ) ;
#34248=CARTESIAN_POINT ( 'NONE',  ( 0.000000000000000000, -20.00000000000000000, 4.899999999999999467 ) ) ;
#34315=AXIS2_PLACEMENT_3D ( 'NONE', #34676, #7985, #8721 ) ;
#34359=ORIENTED_EDGE ( 'NONE', *, *, #17481, .T. ) ;
#34375=CARTESIAN_POINT ( 'NONE',  ( -6.000000000000000888, -30.00000000000000000, -19.99999999999999289 ) ) ;
#34414=EDGE_CURVE ( 'NONE', #9915, #13040, #15367, .T. ) ;
#34451=EDGE_LOOP ( 'NONE', ( #15821, #9999 ) ) ;
#34461=LINE ( 'NONE', #2990, #35224 ) ;
#34555=ORIENTED_EDGE ( 'NONE', *, *, #26990, .T. ) ;
#34571=CARTESIAN_POINT ( 'NONE',  ( 9.184850993605147944E-16, 143.0000000000000000, -7.500000000000000000 ) ) ;
#34610=CARTESIAN_POINT ( 'NONE',  ( 0.000000000000000000, 141.0000000000000000, 0.000000000000000000 ) ) ;
#34676=CARTESIAN_POINT ( 'NONE',  ( 0.000000000000000000, -20.00000000000000000, 0.000000000000000000 ) ) ;
#34764=( NAMED_UNIT ( * ) PLANE_ANGLE_UNIT ( ) SI_UNIT ( $, .RADIAN. ) );
#34827=DIRECTION ( 'NONE',  ( 0.000000000000000000, 1.000000000000000000, 0.000000000000000000 ) ) ;
#34986=VERTEX_POINT ( 'NONE', #27852 ) ;
#35076=DIRECTION ( 'NONE',  ( 1.000000000000000000, 0.000000000000000000, 0.000000000000000000 ) ) ;
#35224=VECTOR ( 'NONE', #19892, 1000.000000000000000 ) ;
#35440=FACE_OUTER_BOUND ( 'NONE', #4270, .T. ) ;
#35479=FACE_BOUND ( 'NONE', #18273, .T. ) ;
#35628=DIRECTION ( 'NONE',  ( 2.168404344971009484E-17, 0.000000000000000000, 1.000000000000000000 ) ) ;
#35662=PLANE ( 'NONE',  #12782 ) ;
#35675=CARTESIAN_POINT ( 'NONE',  ( 0.000000000000000000, 143.0000000000000000, 4.899999999999999467 ) ) ;
#35685=ORIENTED_EDGE ( 'NONE', *, *, #13669, .T. ) ;
#35766=DIRECTION ( 'NONE',  ( 0.000000000000000000, 0.000000000000000000, 1.000000000000000000 ) ) ;
#35781=AXIS2_PLACEMENT_3D ( 'NONE', #10072, #24297, #7054 ) ;
#35796=CARTESIAN_POINT ( 'NONE',  ( 0.000000000000000000, -20.00000000000000000, 4.899999999999999467 ) ) ;
#35907=ADVANCED_BREP_SHAPE_REPRESENTATION ( '', ( #20157, #17215 ), #5638 ) ;
#36039=FACE_BOUND ( 'NONE', #7267, .T. ) ;
#36188=FACE_OUTER_BOUND ( 'NONE', #21951, .T. ) ;
#36290=LINE ( 'NONE', #15846, #27415 ) ;
#36362=CARTESIAN_POINT ( 'NONE',  ( 0.000000000000000000, -20.00000000000000000, 0.000000000000000000 ) ) ;
#36544=AXIS2_PLACEMENT_3D ( 'NONE', #37478, #21015, #11529 ) ;
#36572=CIRCLE ( 'NONE', #16625, 7.500000000000000000 ) ;
#36598=ORIENTED_EDGE ( 'NONE', *, *, #10299, .T. ) ;
#36618=UNCERTAINTY_MEASURE_WITH_UNIT (LENGTH_MEASURE( 1.000000000000000082E-05 ), #6136, 'distance_accuracy_value', 'NONE');
#36759=ORIENTED_EDGE ( 'NONE', *, *, #3459, .F. ) ;
#36787=EDGE_CURVE ( 'NONE', #17895, #5701, #25671, .T. ) ;
#37023=LINE ( 'NONE', #34375, #10546 ) ;
#37207=DIRECTION ( 'NONE',  ( 0.000000000000000000, 1.000000000000000000, 0.000000000000000000 ) ) ;
#37295=DIRECTION ( 'NONE',  ( 0.000000000000000000, 1.000000000000000000, 0.000000000000000000 ) ) ;
#37375=EDGE_CURVE ( 'NONE', #12783, #34986, #36572, .T. ) ;
#37399=EDGE_LOOP ( 'NONE', ( #17569, #3361 ) ) ;
#37478=CARTESIAN_POINT ( 'NONE',  ( 0.000000000000000000, 150.0000000000000000, 0.000000000000000000 ) ) ;
#37529=COLOUR_RGB('Sky Blue',0.24,0.69,0.87);
#37530=FILL_AREA_STYLE_COLOUR('',#37529);
#37531=FILL_AREA_STYLE('',(#37530));
#37532=SURFACE_STYLE_FILL_AREA(#37531);
#37533=SURFACE_SIDE_STYLE('',(#37532));
#37534=SURFACE_STYLE_USAGE(.BOTH.,#37533);
#37535=PRESENTATION_STYLE_ASSIGNMENT((#37534));
ENDSEC;
END-ISO-10303-21;
